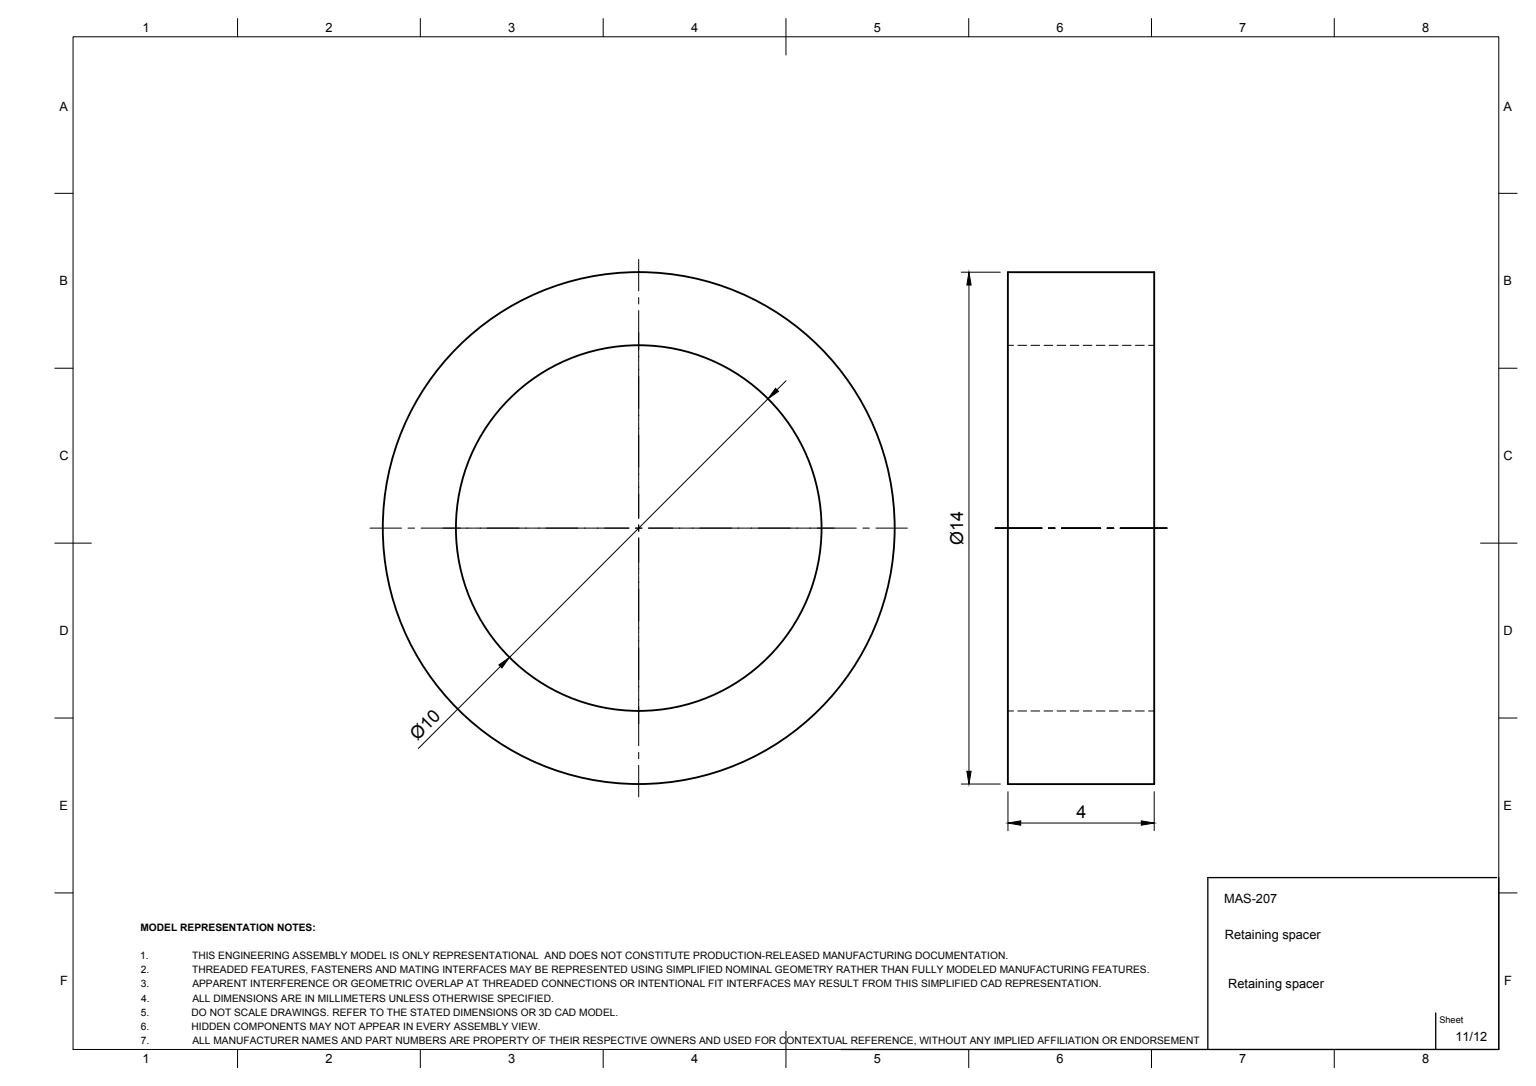
ISO-10303-21;
HEADER;
/* Generated by software containing ST-Developer
 * from STEP Tools, Inc. (www.steptools.com) 
 */

FILE_DESCRIPTION(
/* description */ ('Independent six-slot Geneva indexer. Center distance100, drive radius
50, 60degree indexing per input revolution with120degree engagement an
d240degree dwell. Native machined concave locking faces and relieved d
isk; replaceable retained drive pin; keyed output shaft. Geometry traj
ectory checks use calculated indexing positions, not a contact-dynamic
s simulation. No load or production rating assigned.'),
/* implementation_level */ '2;1');

FILE_NAME(
/* name */ 'Retaining spacer.step',
/* time_stamp */ '2026-11-09T17:53:22-08:00',
/* author */ (''),
/* organization */ (''),
/* preprocessor_version */ 'ST-DEVELOPER v20.2',
/* originating_system */ 'Autodesk Translation Framework v15.17.0.0',
/* authorisation */ '');

FILE_SCHEMA (('AUTOMOTIVE_DESIGN { 1 0 10303 214 3 1 1 }'));
ENDSEC;

DATA;
#10=MECHANICAL_DESIGN_GEOMETRIC_PRESENTATION_REPRESENTATION('',(#109),#4149);
#87=SHAPE_REPRESENTATION_RELATIONSHIP('SRR','None',#4204,#98);
#98=ADVANCED_BREP_SHAPE_REPRESENTATION('',(#120),#4146);
#109=STYLED_ITEM('',(#4266),#120);
#120=MANIFOLD_SOLID_BREP('Body1',#2303);
#157=FACE_BOUND('',#533,.T.);
#158=FACE_BOUND('',#535,.T.);
#230=PLANE('',#2678);
#231=PLANE('',#2679);
#360=FACE_OUTER_BOUND('',#530,.T.);
#361=FACE_OUTER_BOUND('',#531,.T.);
#362=FACE_OUTER_BOUND('',#532,.T.);
#363=FACE_OUTER_BOUND('',#534,.T.);
#530=EDGE_LOOP('',(#2052,#2053,#2054,#2055));
#531=EDGE_LOOP('',(#2056,#2057,#2058,#2059));
#532=EDGE_LOOP('',(#2060));
#533=EDGE_LOOP('',(#2061));
#534=EDGE_LOOP('',(#2062));
#535=EDGE_LOOP('',(#2063));
#708=LINE('',#4055,#880);
#709=LINE('',#4061,#881);
#880=VECTOR('',#3369,5.);
#881=VECTOR('',#3376,7.);
#1004=CIRCLE('',#2673,5.);
#1005=CIRCLE('',#2674,5.);
#1006=CIRCLE('',#2676,7.);
#1007=CIRCLE('',#2677,7.);
#1196=VERTEX_POINT('',#4052);
#1197=VERTEX_POINT('',#4054);
#1198=VERTEX_POINT('',#4058);
#1199=VERTEX_POINT('',#4060);
#1484=EDGE_CURVE('',#1196,#1196,#1004,.T.);
#1485=EDGE_CURVE('',#1196,#1197,#708,.T.);
#1486=EDGE_CURVE('',#1197,#1197,#1005,.T.);
#1487=EDGE_CURVE('',#1198,#1198,#1006,.T.);
#1488=EDGE_CURVE('',#1198,#1199,#709,.T.);
#1489=EDGE_CURVE('',#1199,#1199,#1007,.T.);
#2052=ORIENTED_EDGE('',*,*,#1484,.F.);
#2053=ORIENTED_EDGE('',*,*,#1485,.T.);
#2054=ORIENTED_EDGE('',*,*,#1486,.T.);
#2055=ORIENTED_EDGE('',*,*,#1485,.F.);
#2056=ORIENTED_EDGE('',*,*,#1487,.F.);
#2057=ORIENTED_EDGE('',*,*,#1488,.T.);
#2058=ORIENTED_EDGE('',*,*,#1489,.T.);
#2059=ORIENTED_EDGE('',*,*,#1488,.F.);
#2060=ORIENTED_EDGE('',*,*,#1487,.T.);
#2061=ORIENTED_EDGE('',*,*,#1484,.T.);
#2062=ORIENTED_EDGE('',*,*,#1489,.F.);
#2063=ORIENTED_EDGE('',*,*,#1486,.F.);
#2153=CYLINDRICAL_SURFACE('',#2672,5.);
#2154=CYLINDRICAL_SURFACE('',#2675,7.);
#2281=ADVANCED_FACE('',(#360),#2153,.F.);
#2282=ADVANCED_FACE('',(#361),#2154,.T.);
#2283=ADVANCED_FACE('',(#362,#157),#230,.T.);
#2284=ADVANCED_FACE('',(#363,#158),#231,.F.);
#2303=CLOSED_SHELL('',(#2281,#2282,#2283,#2284));
#2671=AXIS2_PLACEMENT_3D('',#4050,#3363,#3364);
#2672=AXIS2_PLACEMENT_3D('',#4051,#3365,#3366);
#2673=AXIS2_PLACEMENT_3D('',#4053,#3367,#3368);
#2674=AXIS2_PLACEMENT_3D('',#4056,#3370,#3371);
#2675=AXIS2_PLACEMENT_3D('',#4057,#3372,#3373);
#2676=AXIS2_PLACEMENT_3D('',#4059,#3374,#3375);
#2677=AXIS2_PLACEMENT_3D('',#4062,#3377,#3378);
#2678=AXIS2_PLACEMENT_3D('',#4063,#3379,#3380);
#2679=AXIS2_PLACEMENT_3D('',#4064,#3381,#3382);
#3363=DIRECTION('axis',(0.,0.,1.));
#3364=DIRECTION('refdir',(1.,0.,0.));
#3365=DIRECTION('center_axis',(0.,0.,1.));
#3366=DIRECTION('ref_axis',(1.,0.,0.));
#3367=DIRECTION('center_axis',(0.,0.,-1.));
#3368=DIRECTION('ref_axis',(1.,0.,0.));
#3369=DIRECTION('',(0.,0.,-1.));
#3370=DIRECTION('center_axis',(0.,0.,-1.));
#3371=DIRECTION('ref_axis',(1.,0.,0.));
#3372=DIRECTION('center_axis',(0.,0.,1.));
#3373=DIRECTION('ref_axis',(1.,0.,0.));
#3374=DIRECTION('center_axis',(0.,0.,1.));
#3375=DIRECTION('ref_axis',(1.,0.,0.));
#3376=DIRECTION('',(0.,0.,-1.));
#3377=DIRECTION('center_axis',(0.,0.,1.));
#3378=DIRECTION('ref_axis',(1.,0.,0.));
#3379=DIRECTION('center_axis',(0.,0.,1.));
#3380=DIRECTION('ref_axis',(1.,0.,0.));
#3381=DIRECTION('center_axis',(0.,0.,1.));
#3382=DIRECTION('ref_axis',(1.,0.,0.));
#4050=CARTESIAN_POINT('',(0.,0.,0.));
#4051=CARTESIAN_POINT('Origin',(0.,0.,0.));
#4052=CARTESIAN_POINT('',(-5.,-6.12323399573677E-16,4.));
#4053=CARTESIAN_POINT('Origin',(0.,0.,4.));
#4054=CARTESIAN_POINT('',(-5.,-6.12323399573677E-16,0.));
#4055=CARTESIAN_POINT('',(-5.,-6.12323399573677E-16,0.));
#4056=CARTESIAN_POINT('Origin',(0.,0.,0.));
#4057=CARTESIAN_POINT('Origin',(0.,0.,0.));
#4058=CARTESIAN_POINT('',(-7.,-8.57252759403147E-16,4.));
#4059=CARTESIAN_POINT('Origin',(0.,0.,4.));
#4060=CARTESIAN_POINT('',(-7.,-8.57252759403147E-16,0.));
#4061=CARTESIAN_POINT('',(-7.,-8.57252759403147E-16,0.));
#4062=CARTESIAN_POINT('Origin',(0.,0.,0.));
#4063=CARTESIAN_POINT('Origin',(0.,0.,4.));
#4064=CARTESIAN_POINT('Origin',(0.,0.,0.));
#4133=UNCERTAINTY_MEASURE_WITH_UNIT(LENGTH_MEASURE(0.01),#4150,
'DISTANCE_ACCURACY_VALUE',
'Maximum model space distance between geometric entities at asserted c
onnectivities');
#4136=UNCERTAINTY_MEASURE_WITH_UNIT(LENGTH_MEASURE(0.01),#4150,
'DISTANCE_ACCURACY_VALUE',
'Maximum model space distance between geometric entities at asserted c
onnectivities');
#4146=(
GEOMETRIC_REPRESENTATION_CONTEXT(3)
GLOBAL_UNCERTAINTY_ASSIGNED_CONTEXT((#4133))
GLOBAL_UNIT_ASSIGNED_CONTEXT((#4150,#4152,#4153))
REPRESENTATION_CONTEXT('','3D')
);
#4149=(
GEOMETRIC_REPRESENTATION_CONTEXT(3)
GLOBAL_UNCERTAINTY_ASSIGNED_CONTEXT((#4136))
GLOBAL_UNIT_ASSIGNED_CONTEXT((#4150,#4152,#4153))
REPRESENTATION_CONTEXT('','3D')
);
#4150=(
LENGTH_UNIT()
NAMED_UNIT(*)
SI_UNIT(.MILLI.,.METRE.)
);
#4152=(
NAMED_UNIT(*)
PLANE_ANGLE_UNIT()
SI_UNIT($,.RADIAN.)
);
#4153=(
NAMED_UNIT(*)
SI_UNIT($,.STERADIAN.)
SOLID_ANGLE_UNIT()
);
#4163=SHAPE_DEFINITION_REPRESENTATION(#4175,#4204);
#4175=PRODUCT_DEFINITION_SHAPE('',$,#4217);
#4204=SHAPE_REPRESENTATION('',(#2671),#4146);
#4207=PRODUCT_DEFINITION_CONTEXT('part definition',#4245,'design');
#4217=PRODUCT_DEFINITION('Retaining spacer','Retaining spacer',#4229,#4207);
#4229=PRODUCT_DEFINITION_FORMATION('',$,#4256);
#4245=APPLICATION_CONTEXT(
'Core Data for Automotive Mechanical Design Process');
#4246=PRODUCT_CONTEXT('part definition',#4245,'mechanical');
#4256=PRODUCT('Retaining spacer','Retaining spacer',$,(#4246));
#4266=PRESENTATION_STYLE_ASSIGNMENT((#4276));
#4276=SURFACE_STYLE_USAGE(.BOTH.,#4286);
#4286=SURFACE_SIDE_STYLE('',(#4296));
#4296=SURFACE_STYLE_FILL_AREA(#4306);
#4306=FILL_AREA_STYLE('Spacer gray',(#4316));
#4316=FILL_AREA_STYLE_COLOUR('Spacer gray',#4326);
#4326=COLOUR_RGB('Spacer gray',0.407843137254902,0.447058823529412,0.498039215686275);
ENDSEC;
END-ISO-10303-21;
